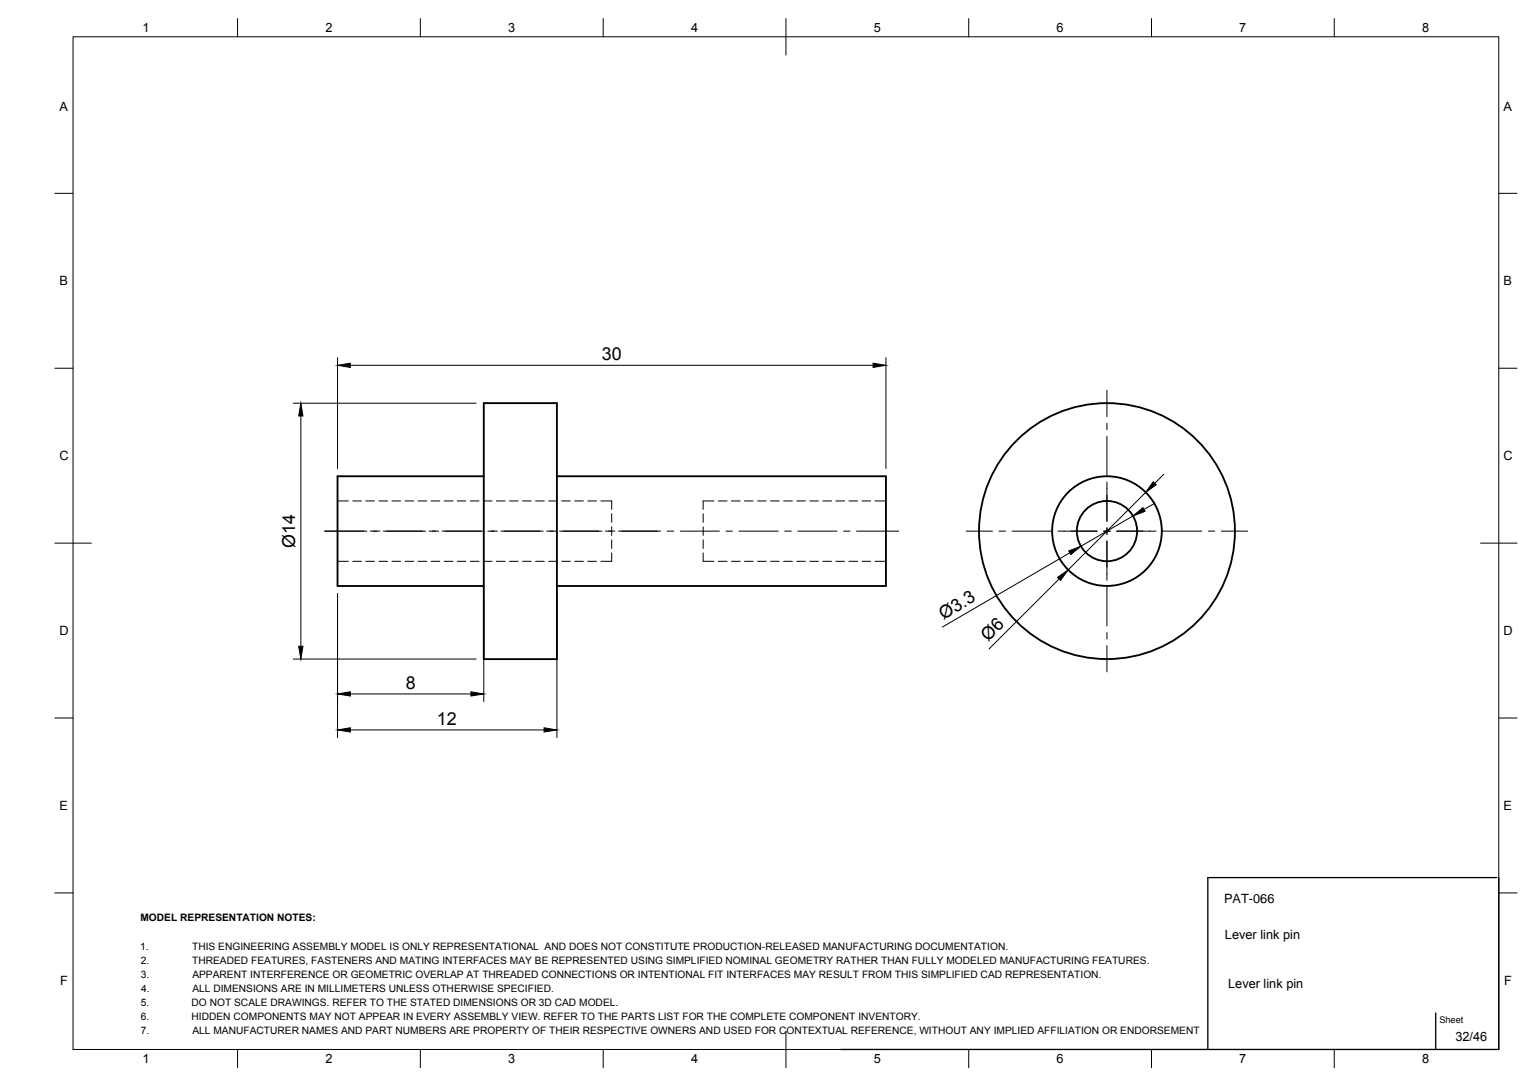
ISO-10303-21;
HEADER;
/* Generated by software containing ST-Developer
 * from STEP Tools, Inc. (www.steptools.com) 
 */

FILE_DESCRIPTION(
/* description */ ('Lever-operated bar clamp (toggle)'),
/* implementation_level */ '2;1');

FILE_NAME(
/* name */ 'Lever link pin.step',
/* time_stamp */ '2026-10-28T03:25:02-07:00',
/* author */ (''),
/* organization */ (''),
/* preprocessor_version */ 'ST-DEVELOPER v20.2',
/* originating_system */ 'Autodesk Translation Framework v15.17.0.0',
/* authorisation */ '');

FILE_SCHEMA (('AUTOMOTIVE_DESIGN { 1 0 10303 214 3 1 1 }'));
ENDSEC;

DATA;
#10=MECHANICAL_DESIGN_GEOMETRIC_PRESENTATION_REPRESENTATION('',(#441),#12413);
#357=SHAPE_REPRESENTATION_RELATIONSHIP('SRR','None',#12599,#395);
#395=ADVANCED_BREP_SHAPE_REPRESENTATION('',(#486),#12396);
#441=STYLED_ITEM('',(#12869),#486);
#486=MANIFOLD_SOLID_BREP('Body1',#6602);
#621=FACE_BOUND('',#1695,.T.);
#622=FACE_BOUND('',#1697,.T.);
#623=FACE_BOUND('',#1702,.T.);
#624=FACE_BOUND('',#1704,.T.);
#802=PLANE('',#7609);
#803=PLANE('',#7613);
#804=PLANE('',#7614);
#805=PLANE('',#7617);
#806=PLANE('',#7625);
#807=PLANE('',#7626);
#1163=FACE_OUTER_BOUND('',#1690,.T.);
#1164=FACE_OUTER_BOUND('',#1691,.T.);
#1165=FACE_OUTER_BOUND('',#1692,.T.);
#1166=FACE_OUTER_BOUND('',#1693,.T.);
#1167=FACE_OUTER_BOUND('',#1694,.T.);
#1168=FACE_OUTER_BOUND('',#1696,.T.);
#1169=FACE_OUTER_BOUND('',#1698,.T.);
#1170=FACE_OUTER_BOUND('',#1699,.T.);
#1171=FACE_OUTER_BOUND('',#1700,.T.);
#1172=FACE_OUTER_BOUND('',#1701,.T.);
#1173=FACE_OUTER_BOUND('',#1703,.T.);
#1690=EDGE_LOOP('',(#5545,#5546,#5547,#5548));
#1691=EDGE_LOOP('',(#5549));
#1692=EDGE_LOOP('',(#5550,#5551,#5552,#5553));
#1693=EDGE_LOOP('',(#5554));
#1694=EDGE_LOOP('',(#5555));
#1695=EDGE_LOOP('',(#5556));
#1696=EDGE_LOOP('',(#5557));
#1697=EDGE_LOOP('',(#5558));
#1698=EDGE_LOOP('',(#5559,#5560,#5561,#5562));
#1699=EDGE_LOOP('',(#5563,#5564,#5565,#5566));
#1700=EDGE_LOOP('',(#5567,#5568,#5569,#5570));
#1701=EDGE_LOOP('',(#5571));
#1702=EDGE_LOOP('',(#5572));
#1703=EDGE_LOOP('',(#5573));
#1704=EDGE_LOOP('',(#5574));
#2135=LINE('',#11702,#2576);
#2136=LINE('',#11709,#2577);
#2137=LINE('',#11723,#2578);
#2138=LINE('',#11726,#2579);
#2139=LINE('',#11731,#2580);
#2576=VECTOR('',#9316,0.165);
#2577=VECTOR('',#9325,0.165);
#2578=VECTOR('',#9344,0.7);
#2579=VECTOR('',#9347,0.3);
#2580=VECTOR('',#9354,0.3);
#2989=CIRCLE('',#7607,0.165);
#2990=CIRCLE('',#7608,0.165);
#2991=CIRCLE('',#7611,0.165);
#2992=CIRCLE('',#7612,0.165);
#2993=CIRCLE('',#7615,0.7);
#2994=CIRCLE('',#7616,0.3);
#2995=CIRCLE('',#7618,0.7);
#2996=CIRCLE('',#7619,0.3);
#2997=CIRCLE('',#7622,0.3);
#2998=CIRCLE('',#7624,0.3);
#3456=VERTEX_POINT('',#11699);
#3457=VERTEX_POINT('',#11701);
#3458=VERTEX_POINT('',#11706);
#3459=VERTEX_POINT('',#11708);
#3460=VERTEX_POINT('',#11713);
#3461=VERTEX_POINT('',#11715);
#3462=VERTEX_POINT('',#11718);
#3463=VERTEX_POINT('',#11720);
#3464=VERTEX_POINT('',#11725);
#3465=VERTEX_POINT('',#11729);
#4177=EDGE_CURVE('',#3456,#3456,#2989,.T.);
#4178=EDGE_CURVE('',#3456,#3457,#2135,.T.);
#4179=EDGE_CURVE('',#3457,#3457,#2990,.T.);
#4180=EDGE_CURVE('',#3458,#3458,#2991,.T.);
#4181=EDGE_CURVE('',#3458,#3459,#2136,.T.);
#4182=EDGE_CURVE('',#3459,#3459,#2992,.T.);
#4183=EDGE_CURVE('',#3460,#3460,#2993,.T.);
#4184=EDGE_CURVE('',#3461,#3461,#2994,.T.);
#4185=EDGE_CURVE('',#3462,#3462,#2995,.T.);
#4186=EDGE_CURVE('',#3463,#3463,#2996,.T.);
#4187=EDGE_CURVE('',#3460,#3462,#2137,.T.);
#4188=EDGE_CURVE('',#3463,#3464,#2138,.T.);
#4189=EDGE_CURVE('',#3464,#3464,#2997,.T.);
#4190=EDGE_CURVE('',#3465,#3465,#2998,.T.);
#4191=EDGE_CURVE('',#3465,#3461,#2139,.T.);
#5545=ORIENTED_EDGE('',*,*,#4177,.F.);
#5546=ORIENTED_EDGE('',*,*,#4178,.T.);
#5547=ORIENTED_EDGE('',*,*,#4179,.F.);
#5548=ORIENTED_EDGE('',*,*,#4178,.F.);
#5549=ORIENTED_EDGE('',*,*,#4177,.T.);
#5550=ORIENTED_EDGE('',*,*,#4180,.F.);
#5551=ORIENTED_EDGE('',*,*,#4181,.T.);
#5552=ORIENTED_EDGE('',*,*,#4182,.T.);
#5553=ORIENTED_EDGE('',*,*,#4181,.F.);
#5554=ORIENTED_EDGE('',*,*,#4182,.F.);
#5555=ORIENTED_EDGE('',*,*,#4183,.T.);
#5556=ORIENTED_EDGE('',*,*,#4184,.F.);
#5557=ORIENTED_EDGE('',*,*,#4185,.F.);
#5558=ORIENTED_EDGE('',*,*,#4186,.F.);
#5559=ORIENTED_EDGE('',*,*,#4183,.F.);
#5560=ORIENTED_EDGE('',*,*,#4187,.T.);
#5561=ORIENTED_EDGE('',*,*,#4185,.T.);
#5562=ORIENTED_EDGE('',*,*,#4187,.F.);
#5563=ORIENTED_EDGE('',*,*,#4186,.T.);
#5564=ORIENTED_EDGE('',*,*,#4188,.T.);
#5565=ORIENTED_EDGE('',*,*,#4189,.T.);
#5566=ORIENTED_EDGE('',*,*,#4188,.F.);
#5567=ORIENTED_EDGE('',*,*,#4190,.F.);
#5568=ORIENTED_EDGE('',*,*,#4191,.T.);
#5569=ORIENTED_EDGE('',*,*,#4184,.T.);
#5570=ORIENTED_EDGE('',*,*,#4191,.F.);
#5571=ORIENTED_EDGE('',*,*,#4190,.T.);
#5572=ORIENTED_EDGE('',*,*,#4179,.T.);
#5573=ORIENTED_EDGE('',*,*,#4189,.F.);
#5574=ORIENTED_EDGE('',*,*,#4180,.T.);
#6128=CYLINDRICAL_SURFACE('',#7606,0.165);
#6129=CYLINDRICAL_SURFACE('',#7610,0.165);
#6130=CYLINDRICAL_SURFACE('',#7620,0.7);
#6131=CYLINDRICAL_SURFACE('',#7621,0.3);
#6132=CYLINDRICAL_SURFACE('',#7623,0.3);
#6438=ADVANCED_FACE('',(#1163),#6128,.F.);
#6439=ADVANCED_FACE('',(#1164),#802,.T.);
#6440=ADVANCED_FACE('',(#1165),#6129,.F.);
#6441=ADVANCED_FACE('',(#1166),#803,.F.);
#6442=ADVANCED_FACE('',(#1167,#621),#804,.T.);
#6443=ADVANCED_FACE('',(#1168,#622),#805,.F.);
#6444=ADVANCED_FACE('',(#1169),#6130,.T.);
#6445=ADVANCED_FACE('',(#1170),#6131,.T.);
#6446=ADVANCED_FACE('',(#1171),#6132,.T.);
#6447=ADVANCED_FACE('',(#1172,#623),#806,.T.);
#6448=ADVANCED_FACE('',(#1173,#624),#807,.F.);
#6602=CLOSED_SHELL('',(#6438,#6439,#6440,#6441,#6442,#6443,#6444,#6445,
#6446,#6447,#6448));
#7605=AXIS2_PLACEMENT_3D('',#11697,#9310,#9311);
#7606=AXIS2_PLACEMENT_3D('',#11698,#9312,#9313);
#7607=AXIS2_PLACEMENT_3D('',#11700,#9314,#9315);
#7608=AXIS2_PLACEMENT_3D('',#11703,#9317,#9318);
#7609=AXIS2_PLACEMENT_3D('',#11704,#9319,#9320);
#7610=AXIS2_PLACEMENT_3D('',#11705,#9321,#9322);
#7611=AXIS2_PLACEMENT_3D('',#11707,#9323,#9324);
#7612=AXIS2_PLACEMENT_3D('',#11710,#9326,#9327);
#7613=AXIS2_PLACEMENT_3D('',#11711,#9328,#9329);
#7614=AXIS2_PLACEMENT_3D('',#11712,#9330,#9331);
#7615=AXIS2_PLACEMENT_3D('',#11714,#9332,#9333);
#7616=AXIS2_PLACEMENT_3D('',#11716,#9334,#9335);
#7617=AXIS2_PLACEMENT_3D('',#11717,#9336,#9337);
#7618=AXIS2_PLACEMENT_3D('',#11719,#9338,#9339);
#7619=AXIS2_PLACEMENT_3D('',#11721,#9340,#9341);
#7620=AXIS2_PLACEMENT_3D('',#11722,#9342,#9343);
#7621=AXIS2_PLACEMENT_3D('',#11724,#9345,#9346);
#7622=AXIS2_PLACEMENT_3D('',#11727,#9348,#9349);
#7623=AXIS2_PLACEMENT_3D('',#11728,#9350,#9351);
#7624=AXIS2_PLACEMENT_3D('',#11730,#9352,#9353);
#7625=AXIS2_PLACEMENT_3D('',#11732,#9355,#9356);
#7626=AXIS2_PLACEMENT_3D('',#11733,#9357,#9358);
#9310=DIRECTION('axis',(0.,0.,1.));
#9311=DIRECTION('refdir',(1.,0.,0.));
#9312=DIRECTION('center_axis',(0.,1.,0.));
#9313=DIRECTION('ref_axis',(1.,0.,0.));
#9314=DIRECTION('center_axis',(0.,1.,0.));
#9315=DIRECTION('ref_axis',(1.,0.,0.));
#9316=DIRECTION('',(0.,1.,0.));
#9317=DIRECTION('center_axis',(0.,-1.,0.));
#9318=DIRECTION('ref_axis',(1.,0.,0.));
#9319=DIRECTION('center_axis',(0.,1.,0.));
#9320=DIRECTION('ref_axis',(1.,0.,0.));
#9321=DIRECTION('center_axis',(0.,1.,0.));
#9322=DIRECTION('ref_axis',(1.,0.,0.));
#9323=DIRECTION('center_axis',(0.,1.,0.));
#9324=DIRECTION('ref_axis',(1.,0.,0.));
#9325=DIRECTION('',(0.,1.,0.));
#9326=DIRECTION('center_axis',(0.,1.,0.));
#9327=DIRECTION('ref_axis',(1.,0.,0.));
#9328=DIRECTION('center_axis',(0.,1.,0.));
#9329=DIRECTION('ref_axis',(1.,0.,0.));
#9330=DIRECTION('center_axis',(0.,1.,0.));
#9331=DIRECTION('ref_axis',(1.,0.,0.));
#9332=DIRECTION('center_axis',(0.,1.,0.));
#9333=DIRECTION('ref_axis',(1.,0.,0.));
#9334=DIRECTION('center_axis',(0.,1.,0.));
#9335=DIRECTION('ref_axis',(1.,0.,0.));
#9336=DIRECTION('center_axis',(0.,1.,0.));
#9337=DIRECTION('ref_axis',(1.,0.,0.));
#9338=DIRECTION('center_axis',(0.,1.,0.));
#9339=DIRECTION('ref_axis',(1.,0.,0.));
#9340=DIRECTION('center_axis',(0.,-1.,0.));
#9341=DIRECTION('ref_axis',(1.,0.,0.));
#9342=DIRECTION('center_axis',(0.,1.,0.));
#9343=DIRECTION('ref_axis',(1.,0.,0.));
#9344=DIRECTION('',(0.,-1.,0.));
#9345=DIRECTION('center_axis',(0.,1.,0.));
#9346=DIRECTION('ref_axis',(1.,0.,0.));
#9347=DIRECTION('',(0.,-1.,0.));
#9348=DIRECTION('center_axis',(0.,1.,0.));
#9349=DIRECTION('ref_axis',(1.,0.,0.));
#9350=DIRECTION('center_axis',(0.,1.,0.));
#9351=DIRECTION('ref_axis',(1.,0.,0.));
#9352=DIRECTION('center_axis',(0.,1.,0.));
#9353=DIRECTION('ref_axis',(1.,0.,0.));
#9354=DIRECTION('',(0.,-1.,0.));
#9355=DIRECTION('center_axis',(0.,1.,0.));
#9356=DIRECTION('ref_axis',(1.,0.,0.));
#9357=DIRECTION('center_axis',(0.,1.,0.));
#9358=DIRECTION('ref_axis',(1.,0.,0.));
#11697=CARTESIAN_POINT('',(0.,0.,0.));
#11698=CARTESIAN_POINT('Origin',(-2.82632109303527,-4.2,8.79263101785268));
#11699=CARTESIAN_POINT('',(-2.99132109303527,-4.2,8.79263101785268));
#11700=CARTESIAN_POINT('Origin',(-2.82632109303527,-4.2,8.79263101785268));
#11701=CARTESIAN_POINT('',(-2.99132109303527,-2.7,8.79263101785268));
#11702=CARTESIAN_POINT('',(-2.99132109303527,-4.2,8.79263101785268));
#11703=CARTESIAN_POINT('Origin',(-2.82632109303527,-2.7,8.79263101785268));
#11704=CARTESIAN_POINT('Origin',(-2.82632109303527,-4.2,8.79263101785268));
#11705=CARTESIAN_POINT('Origin',(-2.82632109303527,-5.8,8.79263101785268));
#11706=CARTESIAN_POINT('',(-2.99132109303527,-5.7,8.79263101785268));
#11707=CARTESIAN_POINT('Origin',(-2.82632109303527,-5.7,8.79263101785268));
#11708=CARTESIAN_POINT('',(-2.99132109303527,-4.7,8.79263101785268));
#11709=CARTESIAN_POINT('',(-2.99132109303527,-5.8,8.79263101785268));
#11710=CARTESIAN_POINT('Origin',(-2.82632109303527,-4.7,8.79263101785268));
#11711=CARTESIAN_POINT('Origin',(-2.82632109303527,-4.7,8.79263101785268));
#11712=CARTESIAN_POINT('Origin',(-2.82632109303527,-3.5,8.79263101785268));
#11713=CARTESIAN_POINT('',(-3.52632109303527,-3.5,8.79263101785268));
#11714=CARTESIAN_POINT('Origin',(-2.82632109303527,-3.5,8.79263101785268));
#11715=CARTESIAN_POINT('',(-3.12632109303527,-3.5,8.79263101785268));
#11716=CARTESIAN_POINT('Origin',(-2.82632109303527,-3.5,8.79263101785268));
#11717=CARTESIAN_POINT('Origin',(-2.82632109303527,-3.9,8.79263101785268));
#11718=CARTESIAN_POINT('',(-3.52632109303527,-3.9,8.79263101785268));
#11719=CARTESIAN_POINT('Origin',(-2.82632109303527,-3.9,8.79263101785268));
#11720=CARTESIAN_POINT('',(-3.12632109303527,-3.9,8.79263101785268));
#11721=CARTESIAN_POINT('Origin',(-2.82632109303527,-3.9,8.79263101785268));
#11722=CARTESIAN_POINT('Origin',(-2.82632109303527,-3.9,8.79263101785268));
#11723=CARTESIAN_POINT('',(-3.52632109303527,-3.9,8.79263101785268));
#11724=CARTESIAN_POINT('Origin',(-2.82632109303527,-5.7,8.79263101785268));
#11725=CARTESIAN_POINT('',(-3.12632109303527,-5.7,8.79263101785268));
#11726=CARTESIAN_POINT('',(-3.12632109303527,-5.7,8.79263101785268));
#11727=CARTESIAN_POINT('Origin',(-2.82632109303527,-5.7,8.79263101785268));
#11728=CARTESIAN_POINT('Origin',(-2.82632109303527,-5.7,8.79263101785268));
#11729=CARTESIAN_POINT('',(-3.12632109303527,-2.7,8.79263101785268));
#11730=CARTESIAN_POINT('Origin',(-2.82632109303527,-2.7,8.79263101785268));
#11731=CARTESIAN_POINT('',(-3.12632109303527,-5.7,8.79263101785268));
#11732=CARTESIAN_POINT('Origin',(-2.82632109303527,-2.7,8.79263101785268));
#11733=CARTESIAN_POINT('Origin',(-2.82632109303527,-5.7,8.79263101785268));
#12350=UNCERTAINTY_MEASURE_WITH_UNIT(LENGTH_MEASURE(0.001),#12414,
'DISTANCE_ACCURACY_VALUE',
'Maximum model space distance between geometric entities at asserted c
onnectivities');
#12367=UNCERTAINTY_MEASURE_WITH_UNIT(LENGTH_MEASURE(0.001),#12414,
'DISTANCE_ACCURACY_VALUE',
'Maximum model space distance between geometric entities at asserted c
onnectivities');
#12396=(
GEOMETRIC_REPRESENTATION_CONTEXT(3)
GLOBAL_UNCERTAINTY_ASSIGNED_CONTEXT((#12350))
GLOBAL_UNIT_ASSIGNED_CONTEXT((#12414,#12416,#12417))
REPRESENTATION_CONTEXT('','3D')
);
#12413=(
GEOMETRIC_REPRESENTATION_CONTEXT(3)
GLOBAL_UNCERTAINTY_ASSIGNED_CONTEXT((#12367))
GLOBAL_UNIT_ASSIGNED_CONTEXT((#12414,#12416,#12417))
REPRESENTATION_CONTEXT('','3D')
);
#12414=(
LENGTH_UNIT()
NAMED_UNIT(*)
SI_UNIT(.CENTI.,.METRE.)
);
#12416=(
NAMED_UNIT(*)
PLANE_ANGLE_UNIT()
SI_UNIT($,.RADIAN.)
);
#12417=(
NAMED_UNIT(*)
SI_UNIT($,.STERADIAN.)
SOLID_ANGLE_UNIT()
);
#12446=SHAPE_DEFINITION_REPRESENTATION(#12498,#12599);
#12498=PRODUCT_DEFINITION_SHAPE('',$,#12645);
#12599=SHAPE_REPRESENTATION('',(#7605),#12396);
#12616=PRODUCT_DEFINITION_CONTEXT('part definition',#12753,'design');
#12645=PRODUCT_DEFINITION('Lever link pin','Lever link pin',#12690,#12616);
#12690=PRODUCT_DEFINITION_FORMATION('',$,#12783);
#12753=APPLICATION_CONTEXT(
'Core Data for Automotive Mechanical Design Process');
#12754=PRODUCT_CONTEXT('part definition',#12753,'mechanical');
#12783=PRODUCT('Lever link pin','Lever link pin','Lever link pin',(#12754));
#12863=COLOUR_RGB('Grey',0.48,0.52,0.57);
#12864=FILL_AREA_STYLE_COLOUR('',#12863);
#12865=FILL_AREA_STYLE('',(#12864));
#12866=SURFACE_STYLE_FILL_AREA(#12865);
#12867=SURFACE_SIDE_STYLE('',(#12866));
#12868=SURFACE_STYLE_USAGE(.BOTH.,#12867);
#12869=PRESENTATION_STYLE_ASSIGNMENT((#12868));
ENDSEC;
END-ISO-10303-21;
